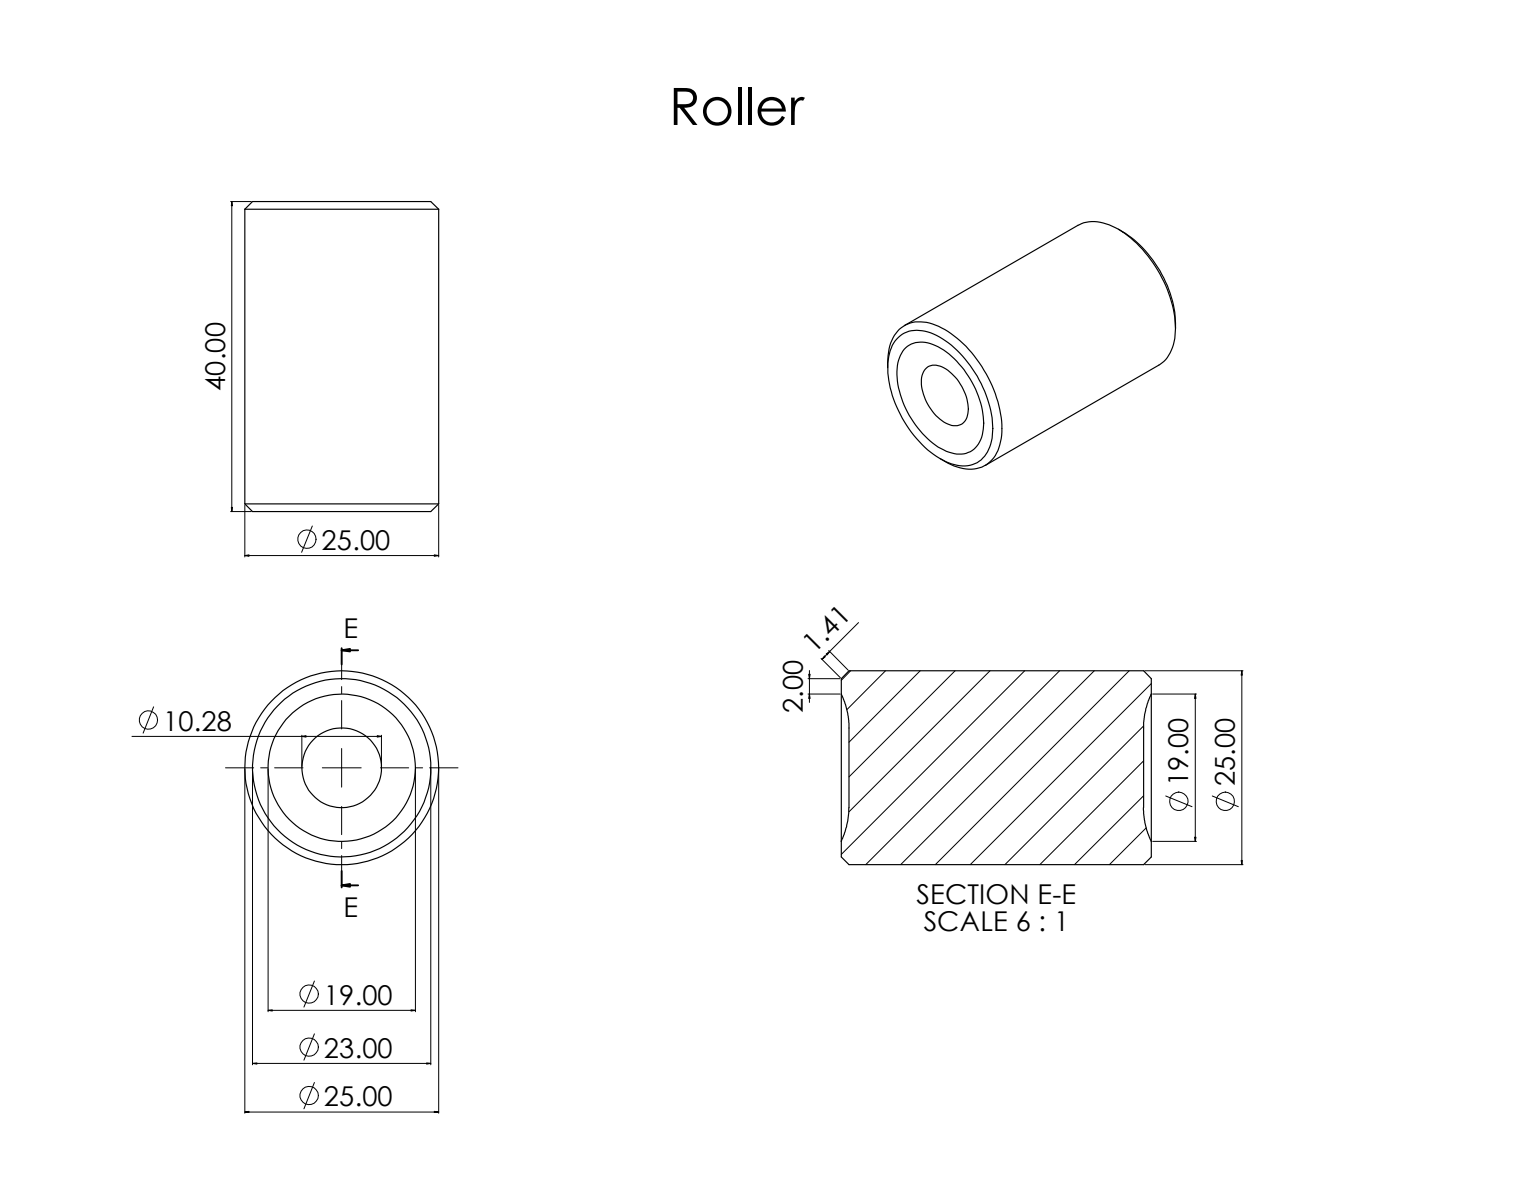
ISO-10303-21;
HEADER;
FILE_DESCRIPTION (('STEP AP214'),
    '1' );
FILE_NAME ('Roller.step',
    '2026-10-25T19:19:31',
    ( '' ),
    ( '' ),
    'SwSTEP 2.0',
    'SolidWorks 2025',
    '' );
FILE_SCHEMA (( 'AUTOMOTIVE_DESIGN' ));
ENDSEC;

DATA;
#23=DIRECTION ( 'NONE',  ( 0.000000000000000000, -1.000000000000000000, 0.000000000000000000 ) ) ;
#60=DIRECTION ( 'NONE',  ( -1.224646799147353207E-16, 1.000000000000000000, 0.000000000000000000 ) ) ;
#62=VECTOR ( 'NONE', #4313, 1000.000000000000000 ) ;
#63=DIRECTION ( 'NONE',  ( 0.000000000000000000, 0.000000000000000000, -1.000000000000000000 ) ) ;
#69=DIRECTION ( 'NONE',  ( -0.000000000000000000, 0.000000000000000000, 1.000000000000000000 ) ) ;
#73=AXIS2_PLACEMENT_3D ( 'NONE', #3304, #3763, #5645 ) ;
#82=SHAPE_REPRESENTATION ( 'Roller', ( #73 ), #2452 ) ;
#83=DIRECTION ( 'NONE',  ( 0.000000000000000000, 0.000000000000000000, 1.000000000000000000 ) ) ;
#94=DIRECTION ( 'NONE',  ( -0.000000000000000000, -0.000000000000000000, -1.000000000000000000 ) ) ;
#98=DIRECTION ( 'NONE',  ( -1.000000000000000000, 0.000000000000000000, 0.000000000000000000 ) ) ;
#101=CARTESIAN_POINT ( 'NONE',  ( 0.000000000000000000, 67.50000000000000000, -20.00000000000000000 ) ) ;
#105=CARTESIAN_POINT ( 'NONE',  ( 0.000000000000000000, 0.000000000000000000, -20.00000000000000000 ) ) ;
#113=LINE ( 'NONE', #4877, #5053 ) ;
#124=CARTESIAN_POINT ( 'NONE',  ( 0.000000000000000000, 67.50000000000000000, -28.99999999999999645 ) ) ;
#134=CARTESIAN_POINT ( 'NONE',  ( 0.000000000000000000, 67.50000000000000000, -19.00000000000000711 ) ) ;
#136=CARTESIAN_POINT ( 'NONE',  ( -5.141101056459331353, 67.50000000000000000, -19.00000000000000000 ) ) ;
#141=DIRECTION ( 'NONE',  ( -1.000000000000000000, 0.000000000000000000, 0.000000000000000000 ) ) ;
#145=EDGE_LOOP ( 'NONE', ( #2402, #588 ) ) ;
#150=DIRECTION ( 'NONE',  ( 0.000000000000000000, 0.000000000000000000, 1.000000000000000000 ) ) ;
#161=APPLICATION_CONTEXT ( 'automotive_design' ) ;
#169=CIRCLE ( 'NONE', #2831, 12.49999999999999822 ) ;
#215=EDGE_CURVE ( 'NONE', #764, #3704, #4242, .T. ) ;
#217=ADVANCED_FACE ( 'NONE', ( #3609 ), #5647, .F. ) ;
#235=CARTESIAN_POINT ( 'NONE',  ( 0.000000000000000000, 67.50000000000000000, 28.99999999999999645 ) ) ;
#266=DIRECTION ( 'NONE',  ( 0.000000000000000000, 0.000000000000000000, -1.000000000000000000 ) ) ;
#285=EDGE_CURVE ( 'NONE', #1194, #1920, #2836, .T. ) ;
#296=CARTESIAN_POINT ( 'NONE',  ( -11.50000000000000355, 67.50000000000000000, 20.00000000000000000 ) ) ;
#305=AXIS2_PLACEMENT_3D ( 'NONE', #991, #5469, #718 ) ;
#318=CARTESIAN_POINT ( 'NONE',  ( 0.000000000000000000, 67.50000000000000000, -19.00000000000000711 ) ) ;
#401=EDGE_CURVE ( 'NONE', #3704, #1698, #113, .T. ) ;
#479=ORIENTED_EDGE ( 'NONE', *, *, #2367, .F. ) ;
#499=ORIENTED_EDGE ( 'NONE', *, *, #5572, .F. ) ;
#513=EDGE_CURVE ( 'NONE', #2290, #1698, #4659, .T. ) ;
#525=EDGE_LOOP ( 'NONE', ( #4665, #4401 ) ) ;
#540=CARTESIAN_POINT ( 'NONE',  ( 0.000000000000000000, 67.50000000000000000, 20.00000000000000000 ) ) ;
#566=AXIS2_PLACEMENT_3D ( 'NONE', #3993, #150, #2542 ) ;
#575=DIRECTION ( 'NONE',  ( 1.000000000000000000, 0.000000000000000000, 0.000000000000000000 ) ) ;
#588=ORIENTED_EDGE ( 'NONE', *, *, #1150, .T. ) ;
#597=ORIENTED_EDGE ( 'NONE', *, *, #5990, .T. ) ;
#598=AXIS2_PLACEMENT_3D ( 'NONE', #1255, #5092, #897 ) ;
#609=TOROIDAL_SURFACE ( 'NONE', #5864, 5.141101056459331353, 10.00000000000000000 ) ;
#618=DIRECTION ( 'NONE',  ( 1.000000000000000000, 0.000000000000000000, 0.000000000000000000 ) ) ;
#643=CARTESIAN_POINT ( 'NONE',  ( 0.000000000000000000, 67.50000000000000000, 20.00000000000000000 ) ) ;
#678=EDGE_LOOP ( 'NONE', ( #3714, #1117 ) ) ;
#695=APPLICATION_CONTEXT ( 'automotive_design' ) ;
#712=ORIENTED_EDGE ( 'NONE', *, *, #2311, .T. ) ;
#718=DIRECTION ( 'NONE',  ( -1.000000000000000000, 0.000000000000000000, 0.000000000000000000 ) ) ;
#731=ORIENTED_EDGE ( 'NONE', *, *, #4522, .T. ) ;
#737=DIRECTION ( 'NONE',  ( -0.000000000000000000, -0.000000000000000000, -1.000000000000000000 ) ) ;
#764=VERTEX_POINT ( 'NONE', #767 ) ;
#767=CARTESIAN_POINT ( 'NONE',  ( -11.50000000000000355, 67.50000000000000000, 20.00000000000000000 ) ) ;
#806=AXIS2_PLACEMENT_3D ( 'NONE', #2341, #23, #1529 ) ;
#810=DIRECTION ( 'NONE',  ( 0.7071067811865489050, 0.000000000000000000, 0.7071067811865462405 ) ) ;
#812=( NAMED_UNIT ( * ) SI_UNIT ( $, .STERADIAN. ) SOLID_ANGLE_UNIT ( ) );
#835=DIRECTION ( 'NONE',  ( 1.000000000000000000, 0.000000000000000000, 0.000000000000000000 ) ) ;
#849=ADVANCED_FACE ( 'NONE', ( #1423, #6132 ), #4314, .F. ) ;
#853=ORIENTED_EDGE ( 'NONE', *, *, #513, .T. ) ;
#859=CIRCLE ( 'NONE', #2034, 11.50000000000000178 ) ;
#884=ADVANCED_FACE ( 'NONE', ( #1985 ), #3751, .T. ) ;
#886=AXIS2_PLACEMENT_3D ( 'NONE', #105, #69, #3322 ) ;
#893=VECTOR ( 'NONE', #5280, 999.9999999999998863 ) ;
#897=DIRECTION ( 'NONE',  ( 1.000000000000000000, 0.000000000000000000, 0.000000000000000000 ) ) ;
#907=DIRECTION ( 'NONE',  ( 1.000000000000000000, 0.000000000000000000, -0.000000000000000000 ) ) ;
#915=VERTEX_POINT ( 'NONE', #1011 ) ;
#927=ORIENTED_EDGE ( 'NONE', *, *, #4966, .F. ) ;
#952=DIRECTION ( 'NONE',  ( 1.000000000000000000, 0.000000000000000000, 0.000000000000000000 ) ) ;
#962=VERTEX_POINT ( 'NONE', #5325 ) ;
#964=CIRCLE ( 'NONE', #5624, 5.141101056459331353 ) ;
#968=ADVANCED_FACE ( 'NONE', ( #1075 ), #3257, .T. ) ;
#991=CARTESIAN_POINT ( 'NONE',  ( 0.000000000000000000, 67.50000000000000000, 20.00000000000000000 ) ) ;
#997=CARTESIAN_POINT ( 'NONE',  ( 0.000000000000000000, 67.50000000000000000, 19.00000000000001066 ) ) ;
#1011=CARTESIAN_POINT ( 'NONE',  ( 12.49999999999999822, 67.50000000000000000, -19.00000000000000711 ) ) ;
#1019=ORIENTED_EDGE ( 'NONE', *, *, #2970, .T. ) ;
#1072=AXIS2_PLACEMENT_3D ( 'NONE', #4812, #2443, #4303 ) ;
#1075=FACE_OUTER_BOUND ( 'NONE', #5391, .T. ) ;
#1094=DIRECTION ( 'NONE',  ( 1.000000000000000000, 0.000000000000000000, 0.000000000000000000 ) ) ;
#1107=AXIS2_PLACEMENT_3D ( 'NONE', #4269, #3765, #952 ) ;
#1117=ORIENTED_EDGE ( 'NONE', *, *, #3706, .F. ) ;
#1150=EDGE_CURVE ( 'NONE', #2322, #6134, #4456, .T. ) ;
#1190=CIRCLE ( 'NONE', #1107, 11.50000000000000355 ) ;
#1192=ORIENTED_EDGE ( 'NONE', *, *, #2118, .F. ) ;
#1194=VERTEX_POINT ( 'NONE', #4324 ) ;
#1241=ORIENTED_EDGE ( 'NONE', *, *, #5676, .F. ) ;
#1254=DIRECTION ( 'NONE',  ( 0.000000000000000000, -0.000000000000000000, -1.000000000000000000 ) ) ;
#1255=CARTESIAN_POINT ( 'NONE',  ( 0.000000000000000000, 67.50000000000000000, 20.00000000000000000 ) ) ;
#1265=PLANE ( 'NONE',  #1544 ) ;
#1282=DIRECTION ( 'NONE',  ( 1.000000000000000000, 0.000000000000000000, 0.000000000000000000 ) ) ;
#1297=ADVANCED_FACE ( 'NONE', ( #2803 ), #609, .F. ) ;
#1321=PRODUCT_DEFINITION_CONTEXT ( 'detailed design', #161, 'design' ) ;
#1339=DIRECTION ( 'NONE',  ( 1.000000000000000000, 0.000000000000000000, 0.000000000000000000 ) ) ;
#1340=DIRECTION ( 'NONE',  ( -1.000000000000000000, 0.000000000000000000, 0.000000000000000000 ) ) ;
#1349=ORIENTED_EDGE ( 'NONE', *, *, #3088, .F. ) ;
#1351=AXIS2_PLACEMENT_3D ( 'NONE', #3508, #4480, #5922 ) ;
#1366=CARTESIAN_POINT ( 'NONE',  ( 0.000000000000000000, 67.50000000000000000, -19.00000000000000711 ) ) ;
#1372=CARTESIAN_POINT ( 'NONE',  ( 0.000000000000000000, 67.50000000000000000, 28.99999999999999645 ) ) ;
#1393=CARTESIAN_POINT ( 'NONE',  ( 0.000000000000000000, 67.50000000000000000, -19.00000000000000000 ) ) ;
#1404=PRODUCT ( 'Roller', 'Roller', '', ( #2650 ) ) ;
#1414=CARTESIAN_POINT ( 'NONE',  ( -5.141101056459331353, 67.50000000000000000, -28.99999999999999645 ) ) ;
#1420=FACE_OUTER_BOUND ( 'NONE', #3483, .T. ) ;
#1423=FACE_BOUND ( 'NONE', #4381, .T. ) ;
#1466=CARTESIAN_POINT ( 'NONE',  ( -12.49999999999999822, 67.50000000000000000, -19.00000000000000711 ) ) ;
#1494=EDGE_CURVE ( 'NONE', #1644, #5747, #1575, .T. ) ;
#1529=DIRECTION ( 'NONE',  ( 0.000000000000000000, 0.000000000000000000, -1.000000000000000000 ) ) ;
#1537=DIRECTION ( 'NONE',  ( 1.224646799147353207E-16, 1.000000000000000000, 0.000000000000000000 ) ) ;
#1544=AXIS2_PLACEMENT_3D ( 'NONE', #4593, #4712, #907 ) ;
#1575=CIRCLE ( 'NONE', #3357, 9.500000000000005329 ) ;
#1579=CYLINDRICAL_SURFACE ( 'NONE', #2668, 12.49999999999999822 ) ;
#1606=VERTEX_POINT ( 'NONE', #6072 ) ;
#1620=CARTESIAN_POINT ( 'NONE',  ( -5.141101056459331353, 67.50000000000000000, 19.00000000000000000 ) ) ;
#1633=EDGE_CURVE ( 'NONE', #2290, #1920, #3384, .T. ) ;
#1644=VERTEX_POINT ( 'NONE', #2658 ) ;
#1698=VERTEX_POINT ( 'NONE', #6130 ) ;
#1710=ORIENTED_EDGE ( 'NONE', *, *, #513, .F. ) ;
#1739=CARTESIAN_POINT ( 'NONE',  ( 0.000000000000000000, 67.50000000000000000, 19.00000000000000000 ) ) ;
#1762=DIRECTION ( 'NONE',  ( 1.000000000000000000, 0.000000000000000000, 0.000000000000000000 ) ) ;
#1801=DIRECTION ( 'NONE',  ( -0.000000000000000000, -0.000000000000000000, -1.000000000000000000 ) ) ;
#1809=FACE_OUTER_BOUND ( 'NONE', #145, .T. ) ;
#1840=ORIENTED_EDGE ( 'NONE', *, *, #2396, .F. ) ;
#1842=PRODUCT_DEFINITION_FORMATION_WITH_SPECIFIED_SOURCE ( 'ANY', '', #1404, .NOT_KNOWN. ) ;
#1868=CARTESIAN_POINT ( 'NONE',  ( 0.000000000000000000, 67.50000000000000000, 20.00000000000000000 ) ) ;
#1894=CARTESIAN_POINT ( 'NONE',  ( 0.000000000000000000, 67.50000000000000000, 20.00000000000000000 ) ) ;
#1900=ORIENTED_EDGE ( 'NONE', *, *, #5035, .F. ) ;
#1920=VERTEX_POINT ( 'NONE', #5795 ) ;
#1947=STYLED_ITEM('',(#6177),#2173);
#1952=DIRECTION ( 'NONE',  ( 0.000000000000000000, 0.000000000000000000, -1.000000000000000000 ) ) ;
#1973=AXIS2_PLACEMENT_3D ( 'NONE', #3459, #266, #5372 ) ;
#1985=FACE_OUTER_BOUND ( 'NONE', #2365, .T. ) ;
#1994=DIRECTION ( 'NONE',  ( 0.7071067811865493491, 8.659560562354955045E-17, -0.7071067811865456854 ) ) ;
#2004=DIRECTION ( 'NONE',  ( 1.000000000000000000, 0.000000000000000000, 0.000000000000000000 ) ) ;
#2019=ORIENTED_EDGE ( 'NONE', *, *, #6136, .T. ) ;
#2034=AXIS2_PLACEMENT_3D ( 'NONE', #3608, #1254, #1339 ) ;
#2053=EDGE_LOOP ( 'NONE', ( #853, #4182, #2832, #4679 ) ) ;
#2083=SHAPE_DEFINITION_REPRESENTATION ( #5686, #82 ) ;
#2086=EDGE_LOOP ( 'NONE', ( #5666, #2334 ) ) ;
#2118=EDGE_CURVE ( 'NONE', #1698, #915, #2449, .T. ) ;
#2165=CIRCLE ( 'NONE', #4867, 11.50000000000000178 ) ;
#2173=MANIFOLD_SOLID_BREP ( 'Fillet1', #5145 ) ;
#2210=DIRECTION ( 'NONE',  ( 1.000000000000000000, 0.000000000000000000, 0.000000000000000000 ) ) ;
#2220=DIRECTION ( 'NONE',  ( -0.000000000000000000, -0.000000000000000000, 1.000000000000000000 ) ) ;
#2228=ORIENTED_EDGE ( 'NONE', *, *, #2759, .F. ) ;
#2229=DIRECTION ( 'NONE',  ( 0.000000000000000000, 0.000000000000000000, 1.000000000000000000 ) ) ;
#2246=VECTOR ( 'NONE', #3017, 1000.000000000000000 ) ;
#2258=CIRCLE ( 'NONE', #5756, 12.49999999999999822 ) ;
#2278=ADVANCED_FACE ( 'NONE', ( #4958 ), #2747, .F. ) ;
#2290=VERTEX_POINT ( 'NONE', #5490 ) ;
#2299=DIRECTION ( 'NONE',  ( -0.000000000000000000, -0.000000000000000000, 1.000000000000000000 ) ) ;
#2305=SHAPE_REPRESENTATION_RELATIONSHIP ( 'NONE' , 'NONE' ,  #82, #6110 ) ;
#2307=( LENGTH_UNIT ( ) NAMED_UNIT ( * ) SI_UNIT ( .MILLI., .METRE. ) );
#2311=EDGE_CURVE ( 'NONE', #1644, #6134, #5736, .T. ) ;
#2322=VERTEX_POINT ( 'NONE', #5461 ) ;
#2324=EDGE_CURVE ( 'NONE', #764, #2290, #4989, .T. ) ;
#2334=ORIENTED_EDGE ( 'NONE', *, *, #3710, .T. ) ;
#2341=CARTESIAN_POINT ( 'NONE',  ( 5.141101056459331353, 67.50000000000000000, -28.99999999999999645 ) ) ;
#2365=EDGE_LOOP ( 'NONE', ( #1019, #2019 ) ) ;
#2367=EDGE_CURVE ( 'NONE', #5096, #962, #5242, .T. ) ;
#2377=CIRCLE ( 'NONE', #806, 10.00000000000000178 ) ;
#2396=EDGE_CURVE ( 'NONE', #962, #5096, #3147, .T. ) ;
#2402=ORIENTED_EDGE ( 'NONE', *, *, #4759, .T. ) ;
#2414=FACE_OUTER_BOUND ( 'NONE', #5765, .T. ) ;
#2431=EDGE_LOOP ( 'NONE', ( #4600, #5834, #5599, #2712 ) ) ;
#2443=DIRECTION ( 'NONE',  ( -0.000000000000000000, -0.000000000000000000, 1.000000000000000000 ) ) ;
#2449=LINE ( 'NONE', #4713, #3446 ) ;
#2452=( GEOMETRIC_REPRESENTATION_CONTEXT ( 3 ) GLOBAL_UNCERTAINTY_ASSIGNED_CONTEXT ( ( #3379 ) ) GLOBAL_UNIT_ASSIGNED_CONTEXT ( ( #6056, #5628, #812 ) ) REPRESENTATION_CONTEXT ( 'NONE', 'WORKASPACE' ) );
#2540=VECTOR ( 'NONE', #810, 999.9999999999998863 ) ;
#2542=DIRECTION ( 'NONE',  ( 1.000000000000000000, 0.000000000000000000, 0.000000000000000000 ) ) ;
#2549=AXIS2_PLACEMENT_3D ( 'NONE', #997, #2880, #1094 ) ;
#2575=AXIS2_PLACEMENT_3D ( 'NONE', #1739, #3641, #1282 ) ;
#2640=ORIENTED_EDGE ( 'NONE', *, *, #1150, .F. ) ;
#2650=PRODUCT_CONTEXT ( 'NONE', #695, 'mechanical' ) ;
#2658=CARTESIAN_POINT ( 'NONE',  ( -9.500000000000008882, 67.50000000000000000, 20.00000000000000000 ) ) ;
#2663=ORIENTED_EDGE ( 'NONE', *, *, #3710, .F. ) ;
#2668=AXIS2_PLACEMENT_3D ( 'NONE', #643, #4410, #3478 ) ;
#2688=ADVANCED_FACE ( 'NONE', ( #1420 ), #1579, .T. ) ;
#2712=ORIENTED_EDGE ( 'NONE', *, *, #5990, .F. ) ;
#2729=AXIS2_PLACEMENT_3D ( 'NONE', #540, #4377, #3445 ) ;
#2747=TOROIDAL_SURFACE ( 'NONE', #3834, 5.141101056459331353, 10.00000000000000000 ) ;
#2759=EDGE_CURVE ( 'NONE', #1920, #915, #2258, .T. ) ;
#2763=DIRECTION ( 'NONE',  ( -0.000000000000000000, -0.000000000000000000, 1.000000000000000000 ) ) ;
#2772=ADVANCED_FACE ( 'NONE', ( #2800, #5113 ), #5175, .T. ) ;
#2776=CARTESIAN_POINT ( 'NONE',  ( 12.49999999999999822, 67.50000000000000000, -19.00000000000000711 ) ) ;
#2793=DIRECTION ( 'NONE',  ( 1.000000000000000000, 0.000000000000000000, 0.000000000000000000 ) ) ;
#2800=FACE_BOUND ( 'NONE', #678, .T. ) ;
#2802=ORIENTED_EDGE ( 'NONE', *, *, #3706, .T. ) ;
#2803=FACE_OUTER_BOUND ( 'NONE', #4809, .T. ) ;
#2831=AXIS2_PLACEMENT_3D ( 'NONE', #318, #2220, #4980 ) ;
#2832=ORIENTED_EDGE ( 'NONE', *, *, #5676, .T. ) ;
#2836=LINE ( 'NONE', #1466, #893 ) ;
#2840=CIRCLE ( 'NONE', #2549, 12.49999999999999822 ) ;
#2880=DIRECTION ( 'NONE',  ( 0.000000000000000000, 0.000000000000000000, -1.000000000000000000 ) ) ;
#2884=FACE_OUTER_BOUND ( 'NONE', #2053, .T. ) ;
#2913=CARTESIAN_POINT ( 'NONE',  ( 0.000000000000000000, 67.50000000000000000, -19.00000000000000000 ) ) ;
#2935=EDGE_CURVE ( 'NONE', #1194, #1606, #2165, .T. ) ;
#2940=AXIS2_PLACEMENT_3D ( 'NONE', #124, #5352, #2004 ) ;
#2955=PRODUCT_DEFINITION ( 'UNKNOWN', '', #1842, #1321 ) ;
#2968=CIRCLE ( 'NONE', #3368, 5.141101056459331353 ) ;
#2970=EDGE_CURVE ( 'NONE', #5318, #3527, #2968, .T. ) ;
#2977=ORIENTED_EDGE ( 'NONE', *, *, #2396, .T. ) ;
#3017=DIRECTION ( 'NONE',  ( -0.7071067811865493491, 0.000000000000000000, -0.7071067811865456854 ) ) ;
#3028=AXIS2_PLACEMENT_3D ( 'NONE', #1894, #3790, #3042 ) ;
#3042=DIRECTION ( 'NONE',  ( -1.000000000000000000, 0.000000000000000000, 0.000000000000000000 ) ) ;
#3071=EDGE_LOOP ( 'NONE', ( #3301, #5846, #4481, #4397 ) ) ;
#3088=EDGE_CURVE ( 'NONE', #962, #5318, #2377, .T. ) ;
#3121=DIRECTION ( 'NONE',  ( -1.000000000000000000, 0.000000000000000000, 0.000000000000000000 ) ) ;
#3122=ORIENTED_EDGE ( 'NONE', *, *, #3088, .T. ) ;
#3125=EDGE_LOOP ( 'NONE', ( #3701, #1840, #3122, #4969 ) ) ;
#3138=ORIENTED_EDGE ( 'NONE', *, *, #2759, .T. ) ;
#3147=CIRCLE ( 'NONE', #5633, 9.500000000000005329 ) ;
#3154=ADVANCED_FACE ( 'NONE', ( #3337 ), #4561, .T. ) ;
#3220=CIRCLE ( 'NONE', #566, 5.141101056459331353 ) ;
#3229=AXIS2_PLACEMENT_3D ( 'NONE', #4307, #60, #98 ) ;
#3257=CONICAL_SURFACE ( 'NONE', #4448, 12.49999999999999822, 0.7853981633974501664 ) ;
#3301=ORIENTED_EDGE ( 'NONE', *, *, #1494, .T. ) ;
#3304=CARTESIAN_POINT ( 'NONE',  ( 0.000000000000000000, 0.000000000000000000, 0.000000000000000000 ) ) ;
#3322=DIRECTION ( 'NONE',  ( 1.000000000000000000, 0.000000000000000000, 0.000000000000000000 ) ) ;
#3337=FACE_OUTER_BOUND ( 'NONE', #2431, .T. ) ;
#3351=DIRECTION ( 'NONE',  ( -1.000000000000000000, 0.000000000000000000, 0.000000000000000000 ) ) ;
#3357=AXIS2_PLACEMENT_3D ( 'NONE', #5492, #2229, #3689 ) ;
#3368=AXIS2_PLACEMENT_3D ( 'NONE', #2913, #63, #3351 ) ;
#3379=UNCERTAINTY_MEASURE_WITH_UNIT (LENGTH_MEASURE( 1.000000000000000082E-05 ), #6056, 'distance_accuracy_value', 'NONE');
#3384=LINE ( 'NONE', #5296, #62 ) ;
#3399=ORIENTED_EDGE ( 'NONE', *, *, #2935, .F. ) ;
#3445=DIRECTION ( 'NONE',  ( -1.000000000000000000, 0.000000000000000000, 0.000000000000000000 ) ) ;
#3446=VECTOR ( 'NONE', #94, 1000.000000000000000 ) ;
#3459=CARTESIAN_POINT ( 'NONE',  ( 0.000000000000000000, 67.50000000000000000, 19.00000000000001066 ) ) ;
#3478=DIRECTION ( 'NONE',  ( -1.000000000000000000, 0.000000000000000000, 0.000000000000000000 ) ) ;
#3483=EDGE_LOOP ( 'NONE', ( #1192, #597, #5167, #3138 ) ) ;
#3508=CARTESIAN_POINT ( 'NONE',  ( -5.141101056459331353, 67.50000000000000000, 28.99999999999999645 ) ) ;
#3527=VERTEX_POINT ( 'NONE', #136 ) ;
#3608=CARTESIAN_POINT ( 'NONE',  ( 0.000000000000000000, 67.50000000000000000, -20.00000000000000000 ) ) ;
#3609=FACE_OUTER_BOUND ( 'NONE', #3071, .T. ) ;
#3637=( GEOMETRIC_REPRESENTATION_CONTEXT ( 3 ) GLOBAL_UNCERTAINTY_ASSIGNED_CONTEXT ( ( #4122 ) ) GLOBAL_UNIT_ASSIGNED_CONTEXT ( ( #2307, #5185, #5335 ) ) REPRESENTATION_CONTEXT ( 'NONE', 'WORKASPACE' ) );
#3641=DIRECTION ( 'NONE',  ( 0.000000000000000000, 0.000000000000000000, 1.000000000000000000 ) ) ;
#3646=AXIS2_PLACEMENT_3D ( 'NONE', #1393, #1952, #5271 ) ;
#3667=DIRECTION ( 'NONE',  ( -0.000000000000000000, 0.000000000000000000, 1.000000000000000000 ) ) ;
#3689=DIRECTION ( 'NONE',  ( 1.000000000000000000, 0.000000000000000000, 0.000000000000000000 ) ) ;
#3701=ORIENTED_EDGE ( 'NONE', *, *, #4522, .F. ) ;
#3704=VERTEX_POINT ( 'NONE', #4703 ) ;
#3706=EDGE_CURVE ( 'NONE', #5747, #1644, #3862, .T. ) ;
#3710=EDGE_CURVE ( 'NONE', #3704, #764, #1190, .T. ) ;
#3714=ORIENTED_EDGE ( 'NONE', *, *, #1494, .F. ) ;
#3746=ORIENTED_EDGE ( 'NONE', *, *, #2324, .F. ) ;
#3751=PLANE ( 'NONE',  #3646 ) ;
#3756=CARTESIAN_POINT ( 'NONE',  ( 0.000000000000000000, 0.000000000000000000, 20.00000000000000000 ) ) ;
#3763=DIRECTION ( 'NONE',  ( 0.000000000000000000, 0.000000000000000000, 1.000000000000000000 ) ) ;
#3765=DIRECTION ( 'NONE',  ( -0.000000000000000000, 0.000000000000000000, 1.000000000000000000 ) ) ;
#3790=DIRECTION ( 'NONE',  ( 0.000000000000000000, 0.000000000000000000, -1.000000000000000000 ) ) ;
#3820=ORIENTED_EDGE ( 'NONE', *, *, #285, .T. ) ;
#3826=AXIS2_PLACEMENT_3D ( 'NONE', #1414, #1537, #5223 ) ;
#3834=AXIS2_PLACEMENT_3D ( 'NONE', #5894, #4005, #3948 ) ;
#3840=AXIS2_PLACEMENT_3D ( 'NONE', #1372, #1801, #1340 ) ;
#3862=CIRCLE ( 'NONE', #4262, 9.500000000000005329 ) ;
#3863=DIRECTION ( 'NONE',  ( 1.000000000000000000, 0.000000000000000000, 0.000000000000000000 ) ) ;
#3899=FACE_OUTER_BOUND ( 'NONE', #3125, .T. ) ;
#3948=DIRECTION ( 'NONE',  ( 1.000000000000000000, 0.000000000000000000, 0.000000000000000000 ) ) ;
#3993=CARTESIAN_POINT ( 'NONE',  ( 0.000000000000000000, 67.50000000000000000, 19.00000000000000000 ) ) ;
#4000=CARTESIAN_POINT ( 'NONE',  ( 5.141101056459331353, 67.50000000000000000, -19.00000000000000000 ) ) ;
#4005=DIRECTION ( 'NONE',  ( -0.000000000000000000, -0.000000000000000000, 1.000000000000000000 ) ) ;
#4017=ORIENTED_EDGE ( 'NONE', *, *, #2367, .T. ) ;
#4094=DIRECTION ( 'NONE',  ( -0.000000000000000000, -0.000000000000000000, 1.000000000000000000 ) ) ;
#4122=UNCERTAINTY_MEASURE_WITH_UNIT (LENGTH_MEASURE( 1.000000000000000082E-05 ), #2307, 'distance_accuracy_value', 'NONE');
#4141=LINE ( 'NONE', #2776, #2540 ) ;
#4182=ORIENTED_EDGE ( 'NONE', *, *, #2118, .T. ) ;
#4213=CIRCLE ( 'NONE', #3229, 10.00000000000000000 ) ;
#4242=CIRCLE ( 'NONE', #598, 11.50000000000000355 ) ;
#4262=AXIS2_PLACEMENT_3D ( 'NONE', #1868, #83, #3863 ) ;
#4269=CARTESIAN_POINT ( 'NONE',  ( 0.000000000000000000, 67.50000000000000000, 20.00000000000000000 ) ) ;
#4303=DIRECTION ( 'NONE',  ( 1.000000000000000000, 0.000000000000000000, 0.000000000000000000 ) ) ;
#4307=CARTESIAN_POINT ( 'NONE',  ( 5.141101056459331353, 67.50000000000000000, 28.99999999999999645 ) ) ;
#4313=DIRECTION ( 'NONE',  ( -0.000000000000000000, -0.000000000000000000, -1.000000000000000000 ) ) ;
#4314=PLANE ( 'NONE',  #886 ) ;
#4324=CARTESIAN_POINT ( 'NONE',  ( -11.50000000000000178, 67.50000000000000000, -20.00000000000000000 ) ) ;
#4372=ADVANCED_FACE ( 'NONE', ( #1809 ), #1265, .T. ) ;
#4377=DIRECTION ( 'NONE',  ( -0.000000000000000000, -0.000000000000000000, -1.000000000000000000 ) ) ;
#4381=EDGE_LOOP ( 'NONE', ( #2977, #4017 ) ) ;
#4397=ORIENTED_EDGE ( 'NONE', *, *, #2311, .F. ) ;
#4401=ORIENTED_EDGE ( 'NONE', *, *, #2935, .T. ) ;
#4410=DIRECTION ( 'NONE',  ( -0.000000000000000000, -0.000000000000000000, -1.000000000000000000 ) ) ;
#4448=AXIS2_PLACEMENT_3D ( 'NONE', #134, #4866, #618 ) ;
#4451=CARTESIAN_POINT ( 'NONE',  ( 0.000000000000000000, 67.50000000000000000, -20.00000000000000000 ) ) ;
#4456=CIRCLE ( 'NONE', #2575, 5.141101056459331353 ) ;
#4480=DIRECTION ( 'NONE',  ( 0.000000000000000000, -1.000000000000000000, 0.000000000000000000 ) ) ;
#4481=ORIENTED_EDGE ( 'NONE', *, *, #4759, .F. ) ;
#4489=ORIENTED_EDGE ( 'NONE', *, *, #2970, .F. ) ;
#4522=EDGE_CURVE ( 'NONE', #5096, #3527, #4623, .T. ) ;
#4537=AXIS2_PLACEMENT_3D ( 'NONE', #4451, #2763, #2793 ) ;
#4561=CONICAL_SURFACE ( 'NONE', #305, 11.50000000000000355, 0.7853981633974509435 ) ;
#4569=ADVANCED_FACE ( 'NONE', ( #3899 ), #5621, .F. ) ;
#4593=CARTESIAN_POINT ( 'NONE',  ( 0.000000000000000000, 67.50000000000000000, 19.00000000000000000 ) ) ;
#4600=ORIENTED_EDGE ( 'NONE', *, *, #401, .F. ) ;
#4623=CIRCLE ( 'NONE', #3826, 9.999999999999998224 ) ;
#4655=EDGE_LOOP ( 'NONE', ( #2663, #5868, #1710, #3746 ) ) ;
#4659=CIRCLE ( 'NONE', #1973, 12.49999999999999822 ) ;
#4664=CARTESIAN_POINT ( 'NONE',  ( 0.000000000000000000, 67.50000000000000000, -20.00000000000000000 ) ) ;
#4665=ORIENTED_EDGE ( 'NONE', *, *, #5035, .T. ) ;
#4679=ORIENTED_EDGE ( 'NONE', *, *, #1633, .F. ) ;
#4703=CARTESIAN_POINT ( 'NONE',  ( 11.50000000000000355, 67.50000000000000000, 20.00000000000000000 ) ) ;
#4712=DIRECTION ( 'NONE',  ( 0.000000000000000000, 0.000000000000000000, 1.000000000000000000 ) ) ;
#4713=CARTESIAN_POINT ( 'NONE',  ( 12.49999999999999822, 67.50000000000000000, 20.00000000000000000 ) ) ;
#4759=EDGE_CURVE ( 'NONE', #6134, #2322, #3220, .T. ) ;
#4787=CYLINDRICAL_SURFACE ( 'NONE', #2729, 12.49999999999999822 ) ;
#4802=FACE_OUTER_BOUND ( 'NONE', #4655, .T. ) ;
#4809=EDGE_LOOP ( 'NONE', ( #499, #2802, #712, #2640 ) ) ;
#4812=CARTESIAN_POINT ( 'NONE',  ( 0.000000000000000000, 67.50000000000000000, -19.00000000000000711 ) ) ;
#4866=DIRECTION ( 'NONE',  ( -0.000000000000000000, -0.000000000000000000, 1.000000000000000000 ) ) ;
#4867=AXIS2_PLACEMENT_3D ( 'NONE', #101, #5724, #575 ) ;
#4877=CARTESIAN_POINT ( 'NONE',  ( 11.50000000000000355, 67.50000000000000000, 20.00000000000000000 ) ) ;
#4941=CARTESIAN_POINT ( 'NONE',  ( 0.000000000000000000, 67.50000000000000000, -19.00000000000000000 ) ) ;
#4957=EDGE_LOOP ( 'NONE', ( #479, #731, #4489, #1349 ) ) ;
#4958=FACE_OUTER_BOUND ( 'NONE', #4957, .T. ) ;
#4966=EDGE_CURVE ( 'NONE', #1606, #915, #4141, .T. ) ;
#4968=AXIS2_PLACEMENT_3D ( 'NONE', #3756, #3667, #2210 ) ;
#4969=ORIENTED_EDGE ( 'NONE', *, *, #6136, .F. ) ;
#4980=DIRECTION ( 'NONE',  ( 1.000000000000000000, 0.000000000000000000, 0.000000000000000000 ) ) ;
#4989=LINE ( 'NONE', #296, #2246 ) ;
#5002=DIRECTION ( 'NONE',  ( 0.000000000000000000, 0.000000000000000000, -1.000000000000000000 ) ) ;
#5035=EDGE_CURVE ( 'NONE', #1606, #1194, #859, .T. ) ;
#5046=MECHANICAL_DESIGN_GEOMETRIC_PRESENTATION_REPRESENTATION('',(#1947),#3637);
#5053=VECTOR ( 'NONE', #1994, 1000.000000000000000 ) ;
#5092=DIRECTION ( 'NONE',  ( -0.000000000000000000, 0.000000000000000000, 1.000000000000000000 ) ) ;
#5096=VERTEX_POINT ( 'NONE', #6080 ) ;
#5113=FACE_OUTER_BOUND ( 'NONE', #2086, .T. ) ;
#5125=CONICAL_SURFACE ( 'NONE', #3028, 11.50000000000000355, 0.7853981633974509435 ) ;
#5132=CONICAL_SURFACE ( 'NONE', #1072, 12.49999999999999822, 0.7853981633974501664 ) ;
#5145=CLOSED_SHELL ( 'NONE', ( #217, #2278, #5227, #968, #5567, #2688, #2772, #849, #6002, #3154, #4372, #884, #4569, #1297 ) ) ;
#5167=ORIENTED_EDGE ( 'NONE', *, *, #1633, .T. ) ;
#5175=PLANE ( 'NONE',  #4968 ) ;
#5185=( NAMED_UNIT ( * ) PLANE_ANGLE_UNIT ( ) SI_UNIT ( $, .RADIAN. ) );
#5189=CARTESIAN_POINT ( 'NONE',  ( 9.500000000000008882, 67.50000000000000000, 20.00000000000000000 ) ) ;
#5223=DIRECTION ( 'NONE',  ( -1.000000000000000000, 0.000000000000000000, 0.000000000000000000 ) ) ;
#5227=ADVANCED_FACE ( 'NONE', ( #4802 ), #5125, .T. ) ;
#5242=CIRCLE ( 'NONE', #4537, 9.500000000000005329 ) ;
#5271=DIRECTION ( 'NONE',  ( 1.000000000000000000, 0.000000000000000000, 0.000000000000000000 ) ) ;
#5280=DIRECTION ( 'NONE',  ( -0.7071067811865489050, 8.659560562354950115E-17, 0.7071067811865462405 ) ) ;
#5296=CARTESIAN_POINT ( 'NONE',  ( -12.49999999999999822, 67.50000000000000000, 20.00000000000000000 ) ) ;
#5318=VERTEX_POINT ( 'NONE', #4000 ) ;
#5325=CARTESIAN_POINT ( 'NONE',  ( 9.500000000000008882, 67.50000000000000000, -20.00000000000000000 ) ) ;
#5335=( NAMED_UNIT ( * ) SI_UNIT ( $, .STERADIAN. ) SOLID_ANGLE_UNIT ( ) );
#5352=DIRECTION ( 'NONE',  ( -0.000000000000000000, -0.000000000000000000, 1.000000000000000000 ) ) ;
#5372=DIRECTION ( 'NONE',  ( 1.000000000000000000, 0.000000000000000000, 0.000000000000000000 ) ) ;
#5391=EDGE_LOOP ( 'NONE', ( #3399, #3820, #1241, #927 ) ) ;
#5461=CARTESIAN_POINT ( 'NONE',  ( 5.141101056459331353, 67.50000000000000000, 19.00000000000000000 ) ) ;
#5469=DIRECTION ( 'NONE',  ( 0.000000000000000000, 0.000000000000000000, -1.000000000000000000 ) ) ;
#5490=CARTESIAN_POINT ( 'NONE',  ( -12.49999999999999822, 67.50000000000000000, 19.00000000000001066 ) ) ;
#5492=CARTESIAN_POINT ( 'NONE',  ( 0.000000000000000000, 67.50000000000000000, 20.00000000000000000 ) ) ;
#5567=ADVANCED_FACE ( 'NONE', ( #2884 ), #4787, .T. ) ;
#5572=EDGE_CURVE ( 'NONE', #5747, #2322, #4213, .T. ) ;
#5599=ORIENTED_EDGE ( 'NONE', *, *, #2324, .T. ) ;
#5621=TOROIDAL_SURFACE ( 'NONE', #2940, 5.141101056459331353, 10.00000000000000000 ) ;
#5624=AXIS2_PLACEMENT_3D ( 'NONE', #4941, #5002, #3121 ) ;
#5628=( NAMED_UNIT ( * ) PLANE_ANGLE_UNIT ( ) SI_UNIT ( $, .RADIAN. ) );
#5633=AXIS2_PLACEMENT_3D ( 'NONE', #4664, #4094, #1762 ) ;
#5645=DIRECTION ( 'NONE',  ( 1.000000000000000000, 0.000000000000000000, 0.000000000000000000 ) ) ;
#5647=TOROIDAL_SURFACE ( 'NONE', #3840, 5.141101056459331353, 10.00000000000000000 ) ;
#5666=ORIENTED_EDGE ( 'NONE', *, *, #215, .T. ) ;
#5676=EDGE_CURVE ( 'NONE', #915, #1920, #169, .T. ) ;
#5686=PRODUCT_DEFINITION_SHAPE ( 'NONE', 'NONE',  #2955 ) ;
#5724=DIRECTION ( 'NONE',  ( 0.000000000000000000, -0.000000000000000000, -1.000000000000000000 ) ) ;
#5736=CIRCLE ( 'NONE', #1351, 10.00000000000000178 ) ;
#5747=VERTEX_POINT ( 'NONE', #5189 ) ;
#5756=AXIS2_PLACEMENT_3D ( 'NONE', #1366, #2299, #835 ) ;
#5765=EDGE_LOOP ( 'NONE', ( #6078, #1900, #6114, #2228 ) ) ;
#5795=CARTESIAN_POINT ( 'NONE',  ( -12.49999999999999822, 67.50000000000000000, -19.00000000000000711 ) ) ;
#5834=ORIENTED_EDGE ( 'NONE', *, *, #215, .F. ) ;
#5846=ORIENTED_EDGE ( 'NONE', *, *, #5572, .T. ) ;
#5864=AXIS2_PLACEMENT_3D ( 'NONE', #235, #737, #141 ) ;
#5868=ORIENTED_EDGE ( 'NONE', *, *, #401, .T. ) ;
#5894=CARTESIAN_POINT ( 'NONE',  ( 0.000000000000000000, 67.50000000000000000, -28.99999999999999645 ) ) ;
#5922=DIRECTION ( 'NONE',  ( 0.000000000000000000, 0.000000000000000000, -1.000000000000000000 ) ) ;
#5990=EDGE_CURVE ( 'NONE', #1698, #2290, #2840, .T. ) ;
#6002=ADVANCED_FACE ( 'NONE', ( #2414 ), #5132, .T. ) ;
#6056=( LENGTH_UNIT ( ) NAMED_UNIT ( * ) SI_UNIT ( .MILLI., .METRE. ) );
#6072=CARTESIAN_POINT ( 'NONE',  ( 11.50000000000000178, 67.50000000000000000, -20.00000000000000000 ) ) ;
#6078=ORIENTED_EDGE ( 'NONE', *, *, #285, .F. ) ;
#6080=CARTESIAN_POINT ( 'NONE',  ( -9.500000000000008882, 67.50000000000000000, -20.00000000000000000 ) ) ;
#6110=ADVANCED_BREP_SHAPE_REPRESENTATION ( '', ( #2173, #73 ), #2452 ) ;
#6114=ORIENTED_EDGE ( 'NONE', *, *, #4966, .T. ) ;
#6130=CARTESIAN_POINT ( 'NONE',  ( 12.49999999999999822, 67.50000000000000000, 19.00000000000001066 ) ) ;
#6132=FACE_OUTER_BOUND ( 'NONE', #525, .T. ) ;
#6134=VERTEX_POINT ( 'NONE', #1620 ) ;
#6136=EDGE_CURVE ( 'NONE', #3527, #5318, #964, .T. ) ;
#6171=COLOUR_RGB('Sky Blue',0.24,0.69,0.87);
#6172=FILL_AREA_STYLE_COLOUR('',#6171);
#6173=FILL_AREA_STYLE('',(#6172));
#6174=SURFACE_STYLE_FILL_AREA(#6173);
#6175=SURFACE_SIDE_STYLE('',(#6174));
#6176=SURFACE_STYLE_USAGE(.BOTH.,#6175);
#6177=PRESENTATION_STYLE_ASSIGNMENT((#6176));
ENDSEC;
END-ISO-10303-21;
